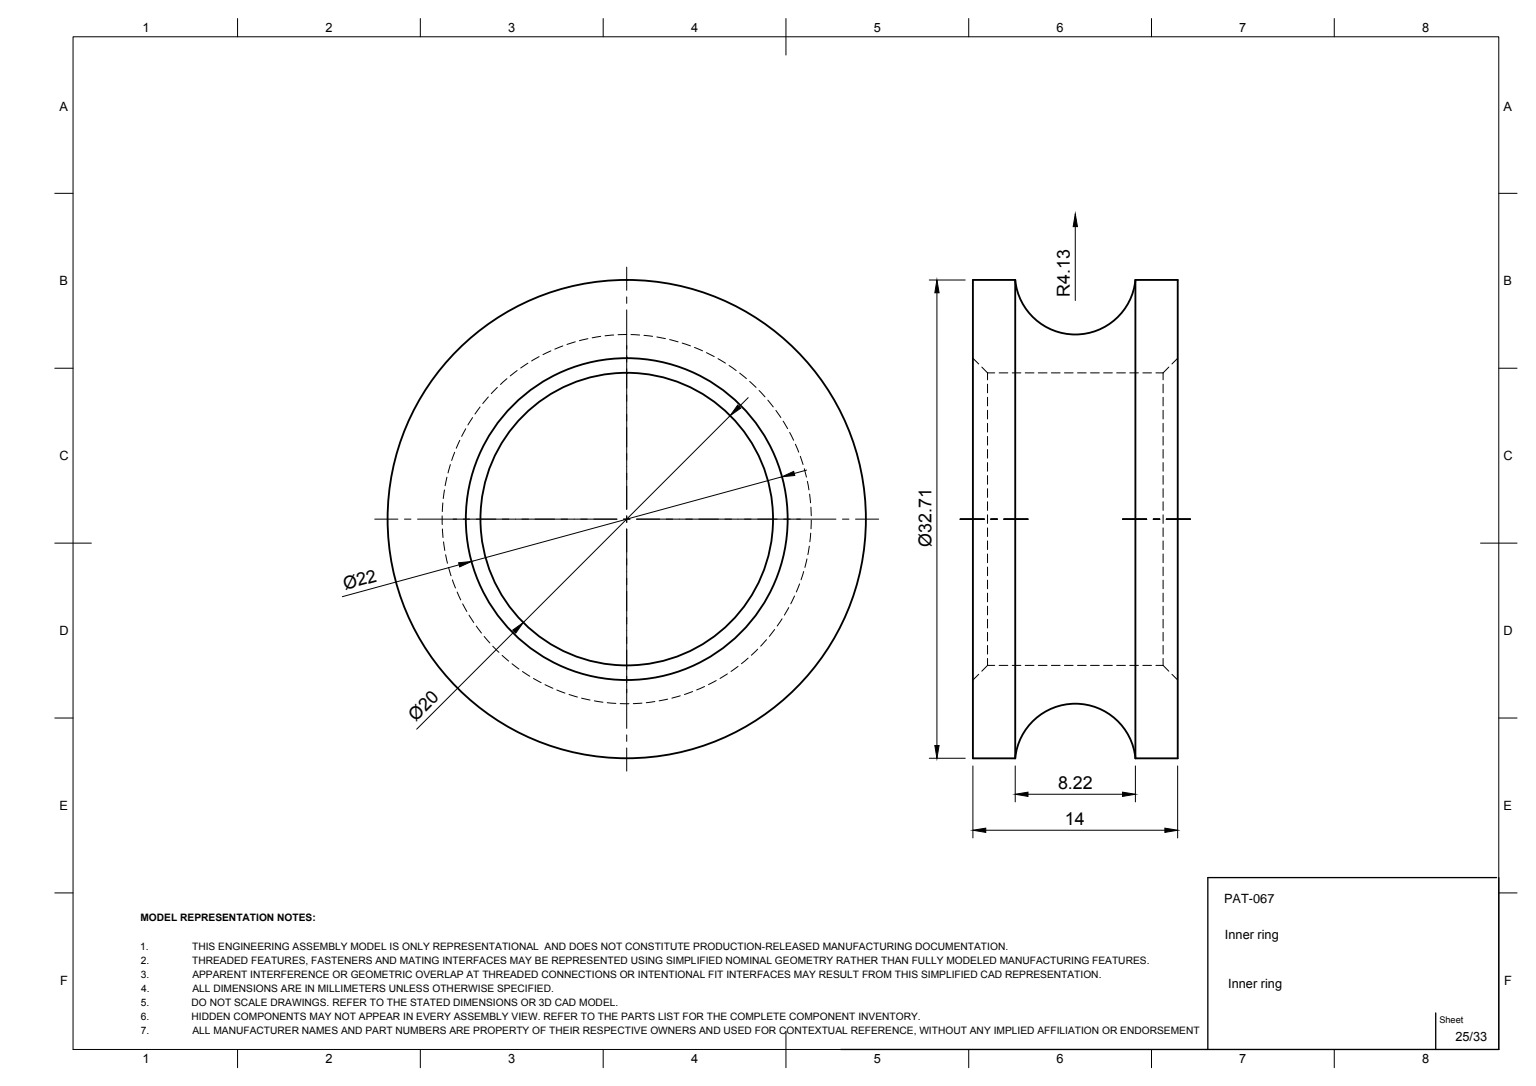
ISO-10303-21;
HEADER;
/* Generated by software containing ST-Developer
 * from STEP Tools, Inc. (www.steptools.com) 
 */

FILE_DESCRIPTION(
/* description */ ('Lifting hook block with sheave'),
/* implementation_level */ '2;1');

FILE_NAME(
/* name */ 'Inner ring.step',
/* time_stamp */ '2026-10-28T03:23:54-07:00',
/* author */ (''),
/* organization */ (''),
/* preprocessor_version */ 'ST-DEVELOPER v20.2',
/* originating_system */ 'Autodesk Translation Framework v15.17.0.0',
/* authorisation */ '');

FILE_SCHEMA (('AUTOMOTIVE_DESIGN { 1 0 10303 214 3 1 1 }'));
ENDSEC;

DATA;
#10=MECHANICAL_DESIGN_GEOMETRIC_PRESENTATION_REPRESENTATION('',(#371),#9391);
#45=TOROIDAL_SURFACE('',#5684,1.675,0.412776);
#278=CONICAL_SURFACE('',#5695,1.05,0.785398163397449);
#279=CONICAL_SURFACE('',#5702,1.05,0.785398163397449);
#311=SHAPE_REPRESENTATION_RELATIONSHIP('SRR','None',#9544,#341);
#341=ADVANCED_BREP_SHAPE_REPRESENTATION('',(#407),#9379);
#371=STYLED_ITEM('',(#9759),#407);
#407=MANIFOLD_SOLID_BREP('Body1',#4909);
#626=LINE('',#8496,#914);
#627=LINE('',#8502,#915);
#628=LINE('',#8506,#916);
#629=LINE('',#8512,#917);
#630=LINE('',#8517,#918);
#914=VECTOR('',#6995,1.63531);
#915=VECTOR('',#7002,1.);
#916=VECTOR('',#7007,1.05);
#917=VECTOR('',#7016,1.63531);
#918=VECTOR('',#7023,1.05);
#1081=CYLINDRICAL_SURFACE('',#5690,1.63531);
#1082=CYLINDRICAL_SURFACE('',#5692,1.);
#1083=CYLINDRICAL_SURFACE('',#5698,1.63531);
#1202=FACE_BOUND('',#1798,.T.);
#1203=FACE_BOUND('',#1801,.T.);
#1409=FACE_OUTER_BOUND('',#1793,.T.);
#1410=FACE_OUTER_BOUND('',#1794,.T.);
#1411=FACE_OUTER_BOUND('',#1795,.T.);
#1412=FACE_OUTER_BOUND('',#1796,.T.);
#1413=FACE_OUTER_BOUND('',#1797,.T.);
#1414=FACE_OUTER_BOUND('',#1799,.T.);
#1415=FACE_OUTER_BOUND('',#1800,.T.);
#1416=FACE_OUTER_BOUND('',#1802,.T.);
#1793=EDGE_LOOP('',(#4034,#4035,#4036,#4037,#4038,#4039));
#1794=EDGE_LOOP('',(#4040,#4041,#4042,#4043,#4044));
#1795=EDGE_LOOP('',(#4045,#4046,#4047,#4048));
#1796=EDGE_LOOP('',(#4049,#4050,#4051,#4052));
#1797=EDGE_LOOP('',(#4053));
#1798=EDGE_LOOP('',(#4054));
#1799=EDGE_LOOP('',(#4055,#4056,#4057,#4058,#4059));
#1800=EDGE_LOOP('',(#4060));
#1801=EDGE_LOOP('',(#4061));
#1802=EDGE_LOOP('',(#4062,#4063,#4064,#4065));
#2103=CIRCLE('',#5685,1.63531);
#2104=CIRCLE('',#5686,1.63531);
#2105=CIRCLE('',#5687,0.412776);
#2106=CIRCLE('',#5688,1.63531);
#2107=CIRCLE('',#5689,1.63531);
#2108=CIRCLE('',#5691,1.63531);
#2109=CIRCLE('',#5693,1.);
#2110=CIRCLE('',#5694,1.);
#2111=CIRCLE('',#5696,1.1);
#2112=CIRCLE('',#5699,1.63531);
#2113=CIRCLE('',#5701,1.1);
#2472=VERTEX_POINT('',#8485);
#2473=VERTEX_POINT('',#8486);
#2474=VERTEX_POINT('',#8489);
#2475=VERTEX_POINT('',#8491);
#2476=VERTEX_POINT('',#8495);
#2477=VERTEX_POINT('',#8499);
#2478=VERTEX_POINT('',#8501);
#2479=VERTEX_POINT('',#8505);
#2480=VERTEX_POINT('',#8510);
#2481=VERTEX_POINT('',#8514);
#3021=EDGE_CURVE('',#2472,#2473,#2103,.T.);
#3022=EDGE_CURVE('',#2473,#2472,#2104,.T.);
#3023=EDGE_CURVE('',#2473,#2474,#2105,.T.);
#3024=EDGE_CURVE('',#2475,#2474,#2106,.T.);
#3025=EDGE_CURVE('',#2474,#2475,#2107,.T.);
#3026=EDGE_CURVE('',#2475,#2476,#626,.T.);
#3027=EDGE_CURVE('',#2476,#2476,#2108,.T.);
#3028=EDGE_CURVE('',#2477,#2477,#2109,.T.);
#3029=EDGE_CURVE('',#2477,#2478,#627,.T.);
#3030=EDGE_CURVE('',#2478,#2478,#2110,.T.);
#3031=EDGE_CURVE('',#2478,#2479,#628,.T.);
#3032=EDGE_CURVE('',#2479,#2479,#2111,.T.);
#3033=EDGE_CURVE('',#2480,#2480,#2112,.T.);
#3034=EDGE_CURVE('',#2480,#2472,#629,.T.);
#3035=EDGE_CURVE('',#2481,#2481,#2113,.T.);
#3036=EDGE_CURVE('',#2481,#2477,#630,.T.);
#4034=ORIENTED_EDGE('',*,*,#3021,.F.);
#4035=ORIENTED_EDGE('',*,*,#3022,.F.);
#4036=ORIENTED_EDGE('',*,*,#3023,.T.);
#4037=ORIENTED_EDGE('',*,*,#3024,.F.);
#4038=ORIENTED_EDGE('',*,*,#3025,.F.);
#4039=ORIENTED_EDGE('',*,*,#3023,.F.);
#4040=ORIENTED_EDGE('',*,*,#3024,.T.);
#4041=ORIENTED_EDGE('',*,*,#3025,.T.);
#4042=ORIENTED_EDGE('',*,*,#3026,.T.);
#4043=ORIENTED_EDGE('',*,*,#3027,.T.);
#4044=ORIENTED_EDGE('',*,*,#3026,.F.);
#4045=ORIENTED_EDGE('',*,*,#3028,.T.);
#4046=ORIENTED_EDGE('',*,*,#3029,.T.);
#4047=ORIENTED_EDGE('',*,*,#3030,.F.);
#4048=ORIENTED_EDGE('',*,*,#3029,.F.);
#4049=ORIENTED_EDGE('',*,*,#3030,.T.);
#4050=ORIENTED_EDGE('',*,*,#3031,.T.);
#4051=ORIENTED_EDGE('',*,*,#3032,.F.);
#4052=ORIENTED_EDGE('',*,*,#3031,.F.);
#4053=ORIENTED_EDGE('',*,*,#3027,.F.);
#4054=ORIENTED_EDGE('',*,*,#3032,.T.);
#4055=ORIENTED_EDGE('',*,*,#3033,.F.);
#4056=ORIENTED_EDGE('',*,*,#3034,.T.);
#4057=ORIENTED_EDGE('',*,*,#3021,.T.);
#4058=ORIENTED_EDGE('',*,*,#3022,.T.);
#4059=ORIENTED_EDGE('',*,*,#3034,.F.);
#4060=ORIENTED_EDGE('',*,*,#3033,.T.);
#4061=ORIENTED_EDGE('',*,*,#3035,.F.);
#4062=ORIENTED_EDGE('',*,*,#3035,.T.);
#4063=ORIENTED_EDGE('',*,*,#3036,.T.);
#4064=ORIENTED_EDGE('',*,*,#3028,.F.);
#4065=ORIENTED_EDGE('',*,*,#3036,.F.);
#4547=PLANE('',#5697);
#4548=PLANE('',#5700);
#4785=ADVANCED_FACE('',(#1409),#45,.F.);
#4786=ADVANCED_FACE('',(#1410),#1081,.T.);
#4787=ADVANCED_FACE('',(#1411),#1082,.F.);
#4788=ADVANCED_FACE('',(#1412),#278,.F.);
#4789=ADVANCED_FACE('',(#1413,#1202),#4547,.T.);
#4790=ADVANCED_FACE('',(#1414),#1083,.T.);
#4791=ADVANCED_FACE('',(#1415,#1203),#4548,.T.);
#4792=ADVANCED_FACE('',(#1416),#279,.F.);
#4909=CLOSED_SHELL('',(#4785,#4786,#4787,#4788,#4789,#4790,#4791,#4792));
#5683=AXIS2_PLACEMENT_3D('',#8483,#6979,#6980);
#5684=AXIS2_PLACEMENT_3D('',#8484,#6981,#6982);
#5685=AXIS2_PLACEMENT_3D('',#8487,#6983,#6984);
#5686=AXIS2_PLACEMENT_3D('',#8488,#6985,#6986);
#5687=AXIS2_PLACEMENT_3D('',#8490,#6987,#6988);
#5688=AXIS2_PLACEMENT_3D('',#8492,#6989,#6990);
#5689=AXIS2_PLACEMENT_3D('',#8493,#6991,#6992);
#5690=AXIS2_PLACEMENT_3D('',#8494,#6993,#6994);
#5691=AXIS2_PLACEMENT_3D('',#8497,#6996,#6997);
#5692=AXIS2_PLACEMENT_3D('',#8498,#6998,#6999);
#5693=AXIS2_PLACEMENT_3D('',#8500,#7000,#7001);
#5694=AXIS2_PLACEMENT_3D('',#8503,#7003,#7004);
#5695=AXIS2_PLACEMENT_3D('',#8504,#7005,#7006);
#5696=AXIS2_PLACEMENT_3D('',#8507,#7008,#7009);
#5697=AXIS2_PLACEMENT_3D('',#8508,#7010,#7011);
#5698=AXIS2_PLACEMENT_3D('',#8509,#7012,#7013);
#5699=AXIS2_PLACEMENT_3D('',#8511,#7014,#7015);
#5700=AXIS2_PLACEMENT_3D('',#8513,#7017,#7018);
#5701=AXIS2_PLACEMENT_3D('',#8515,#7019,#7020);
#5702=AXIS2_PLACEMENT_3D('',#8516,#7021,#7022);
#6979=DIRECTION('axis',(0.,0.,1.));
#6980=DIRECTION('refdir',(1.,0.,0.));
#6981=DIRECTION('center_axis',(0.,-1.,0.));
#6982=DIRECTION('ref_axis',(0.,0.,-1.));
#6983=DIRECTION('center_axis',(0.,-1.,0.));
#6984=DIRECTION('ref_axis',(1.,0.,0.));
#6985=DIRECTION('center_axis',(0.,-1.,0.));
#6986=DIRECTION('ref_axis',(1.,0.,0.));
#6987=DIRECTION('center_axis',(1.,0.,1.22464679914735E-16));
#6988=DIRECTION('ref_axis',(-1.22464679914735E-16,0.,1.));
#6989=DIRECTION('center_axis',(0.,1.,0.));
#6990=DIRECTION('ref_axis',(1.,0.,0.));
#6991=DIRECTION('center_axis',(0.,1.,0.));
#6992=DIRECTION('ref_axis',(1.,0.,0.));
#6993=DIRECTION('center_axis',(0.,-1.,0.));
#6994=DIRECTION('ref_axis',(1.,0.,0.));
#6995=DIRECTION('',(0.,1.,0.));
#6996=DIRECTION('center_axis',(0.,-1.,0.));
#6997=DIRECTION('ref_axis',(1.,0.,0.));
#6998=DIRECTION('center_axis',(0.,-1.,0.));
#6999=DIRECTION('ref_axis',(1.,0.,0.));
#7000=DIRECTION('center_axis',(0.,-1.,0.));
#7001=DIRECTION('ref_axis',(1.,0.,0.));
#7002=DIRECTION('',(0.,1.,0.));
#7003=DIRECTION('center_axis',(0.,-1.,0.));
#7004=DIRECTION('ref_axis',(1.,0.,0.));
#7005=DIRECTION('center_axis',(0.,1.,0.));
#7006=DIRECTION('ref_axis',(1.,0.,0.));
#7007=DIRECTION('',(-0.707106781186548,0.707106781186547,-8.65956056235494E-17));
#7008=DIRECTION('center_axis',(0.,-1.,0.));
#7009=DIRECTION('ref_axis',(1.,0.,0.));
#7010=DIRECTION('center_axis',(0.,1.,0.));
#7011=DIRECTION('ref_axis',(0.,0.,1.));
#7012=DIRECTION('center_axis',(0.,-1.,0.));
#7013=DIRECTION('ref_axis',(1.,0.,0.));
#7014=DIRECTION('center_axis',(0.,-1.,0.));
#7015=DIRECTION('ref_axis',(1.,0.,0.));
#7016=DIRECTION('',(0.,1.,0.));
#7017=DIRECTION('center_axis',(0.,-1.,0.));
#7018=DIRECTION('ref_axis',(0.,0.,-1.));
#7019=DIRECTION('center_axis',(0.,-1.,0.));
#7020=DIRECTION('ref_axis',(1.,0.,0.));
#7021=DIRECTION('center_axis',(0.,-1.,0.));
#7022=DIRECTION('ref_axis',(1.,0.,0.));
#7023=DIRECTION('',(0.707106781186548,0.707106781186547,8.65956056235494E-17));
#8483=CARTESIAN_POINT('',(0.,0.,0.));
#8484=CARTESIAN_POINT('Origin',(0.,0.,0.));
#8485=CARTESIAN_POINT('',(-1.63531,-0.410863395882378,-2.00267715711366E-16));
#8486=CARTESIAN_POINT('',(-2.00267715711366E-16,-0.410863395882378,1.63531));
#8487=CARTESIAN_POINT('Origin',(0.,-0.410863395882378,0.));
#8488=CARTESIAN_POINT('Origin',(0.,-0.410863395882378,0.));
#8489=CARTESIAN_POINT('',(-2.00267715711366E-16,0.410863395882378,1.63531));
#8490=CARTESIAN_POINT('Origin',(-2.05128338857182E-16,0.,1.675));
#8491=CARTESIAN_POINT('',(-1.63531,0.410863395882378,2.00267715711366E-16));
#8492=CARTESIAN_POINT('Origin',(0.,0.410863395882378,0.));
#8493=CARTESIAN_POINT('Origin',(0.,0.410863395882378,0.));
#8494=CARTESIAN_POINT('Origin',(0.,0.,0.));
#8495=CARTESIAN_POINT('',(-1.63531,0.7,-2.00267715711366E-16));
#8496=CARTESIAN_POINT('',(-1.63531,0.,-2.00267715711366E-16));
#8497=CARTESIAN_POINT('Origin',(0.,0.7,0.));
#8498=CARTESIAN_POINT('Origin',(0.,0.,0.));
#8499=CARTESIAN_POINT('',(-1.,-0.6,-1.22464679914735E-16));
#8500=CARTESIAN_POINT('Origin',(0.,-0.6,0.));
#8501=CARTESIAN_POINT('',(-1.,0.6,-1.22464679914735E-16));
#8502=CARTESIAN_POINT('',(-1.,0.,-1.22464679914735E-16));
#8503=CARTESIAN_POINT('Origin',(0.,0.6,0.));
#8504=CARTESIAN_POINT('Origin',(0.,0.65,0.));
#8505=CARTESIAN_POINT('',(-1.1,0.7,-1.34711147906209E-16));
#8506=CARTESIAN_POINT('',(-1.05,0.65,-1.28587913910472E-16));
#8507=CARTESIAN_POINT('Origin',(0.,0.7,0.));
#8508=CARTESIAN_POINT('Origin',(1.63531,0.7,0.));
#8509=CARTESIAN_POINT('Origin',(0.,0.,0.));
#8510=CARTESIAN_POINT('',(-1.63531,-0.7,-2.00267715711366E-16));
#8511=CARTESIAN_POINT('Origin',(0.,-0.7,0.));
#8512=CARTESIAN_POINT('',(-1.63531,0.,-2.00267715711366E-16));
#8513=CARTESIAN_POINT('Origin',(1.1,-0.7,0.));
#8514=CARTESIAN_POINT('',(-1.1,-0.7,-1.34711147906209E-16));
#8515=CARTESIAN_POINT('Origin',(0.,-0.7,0.));
#8516=CARTESIAN_POINT('Origin',(0.,-0.65,0.));
#8517=CARTESIAN_POINT('',(-1.05,-0.65,-1.28587913910472E-16));
#9342=UNCERTAINTY_MEASURE_WITH_UNIT(LENGTH_MEASURE(0.001),#9392,
'DISTANCE_ACCURACY_VALUE',
'Maximum model space distance between geometric entities at asserted c
onnectivities');
#9354=UNCERTAINTY_MEASURE_WITH_UNIT(LENGTH_MEASURE(0.001),#9392,
'DISTANCE_ACCURACY_VALUE',
'Maximum model space distance between geometric entities at asserted c
onnectivities');
#9379=(
GEOMETRIC_REPRESENTATION_CONTEXT(3)
GLOBAL_UNCERTAINTY_ASSIGNED_CONTEXT((#9342))
GLOBAL_UNIT_ASSIGNED_CONTEXT((#9392,#9394,#9395))
REPRESENTATION_CONTEXT('','3D')
);
#9391=(
GEOMETRIC_REPRESENTATION_CONTEXT(3)
GLOBAL_UNCERTAINTY_ASSIGNED_CONTEXT((#9354))
GLOBAL_UNIT_ASSIGNED_CONTEXT((#9392,#9394,#9395))
REPRESENTATION_CONTEXT('','3D')
);
#9392=(
LENGTH_UNIT()
NAMED_UNIT(*)
SI_UNIT(.CENTI.,.METRE.)
);
#9394=(
NAMED_UNIT(*)
PLANE_ANGLE_UNIT()
SI_UNIT($,.RADIAN.)
);
#9395=(
NAMED_UNIT(*)
SI_UNIT($,.STERADIAN.)
SOLID_ANGLE_UNIT()
);
#9420=SHAPE_DEFINITION_REPRESENTATION(#9481,#9544);
#9481=PRODUCT_DEFINITION_SHAPE('',$,#9581);
#9544=SHAPE_REPRESENTATION('',(#5683),#9379);
#9556=PRODUCT_DEFINITION_CONTEXT('part definition',#9666,'design');
#9581=PRODUCT_DEFINITION('Inner ring','Inner ring',#9617,#9556);
#9617=PRODUCT_DEFINITION_FORMATION('',$,#9692);
#9666=APPLICATION_CONTEXT(
'Core Data for Automotive Mechanical Design Process');
#9667=PRODUCT_CONTEXT('part definition',#9666,'mechanical');
#9692=PRODUCT('Inner ring','Inner ring','Inner ring',(#9667));
#9753=COLOUR_RGB('Grey',0.48,0.52,0.57);
#9754=FILL_AREA_STYLE_COLOUR('',#9753);
#9755=FILL_AREA_STYLE('',(#9754));
#9756=SURFACE_STYLE_FILL_AREA(#9755);
#9757=SURFACE_SIDE_STYLE('',(#9756));
#9758=SURFACE_STYLE_USAGE(.BOTH.,#9757);
#9759=PRESENTATION_STYLE_ASSIGNMENT((#9758));
ENDSEC;
END-ISO-10303-21;
